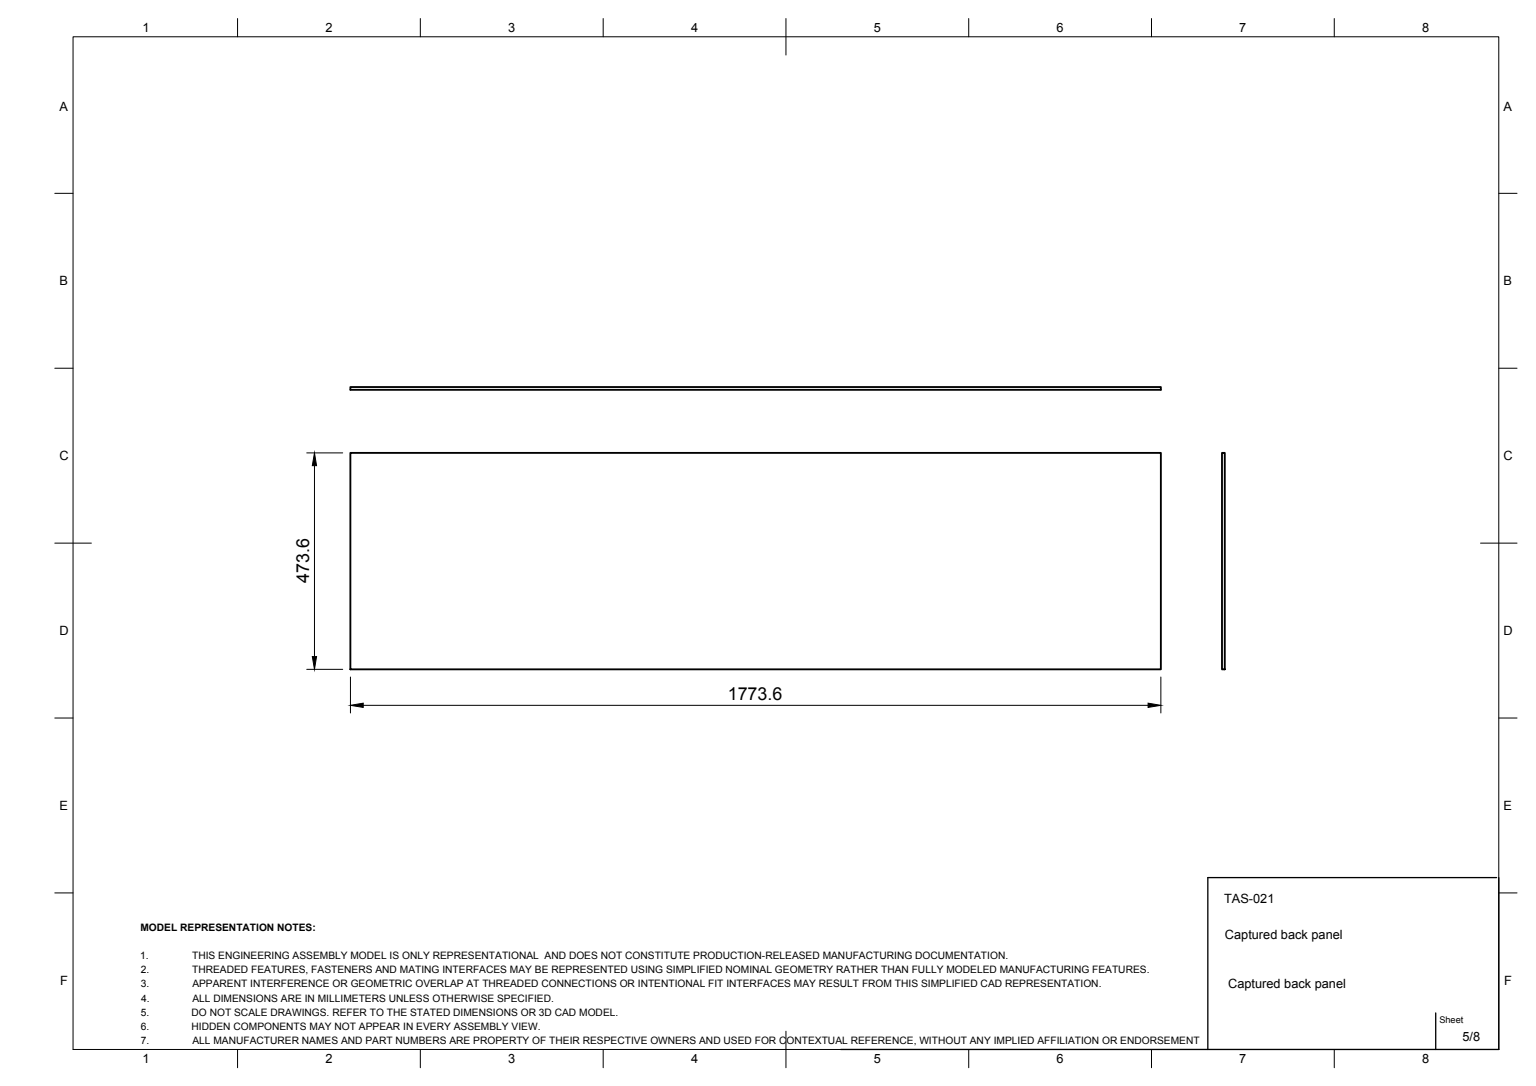
ISO-10303-21;
HEADER;
/* Generated by software containing ST-Developer
 * from STEP Tools, Inc. (www.steptools.com) 
 */

FILE_DESCRIPTION(
/* description */ (''),
/* implementation_level */ '2;1');

FILE_NAME(
/* name */ 'Captured back panel.step',
/* time_stamp */ '2026-11-15T17:48:08-08:00',
/* author */ (''),
/* organization */ (''),
/* preprocessor_version */ 'ST-DEVELOPER v20.2',
/* originating_system */ 'Autodesk Translation Framework v15.17.0.0',
/* authorisation */ '');

FILE_SCHEMA (('AUTOMOTIVE_DESIGN { 1 0 10303 214 3 1 1 }'));
ENDSEC;

DATA;
#10=MECHANICAL_DESIGN_GEOMETRIC_PRESENTATION_REPRESENTATION('',(#141),#2097);
#129=SHAPE_REPRESENTATION_RELATIONSHIP('SRR','None',#2148,#135);
#135=ADVANCED_BREP_SHAPE_REPRESENTATION('',(#147),#2093);
#141=STYLED_ITEM('',(#2187),#147);
#147=MANIFOLD_SOLID_BREP('Body1',#1195);
#197=PLANE('',#1326);
#198=PLANE('',#1327);
#199=PLANE('',#1328);
#200=PLANE('',#1329);
#201=PLANE('',#1330);
#202=PLANE('',#1331);
#259=FACE_OUTER_BOUND('',#331,.T.);
#260=FACE_OUTER_BOUND('',#332,.T.);
#261=FACE_OUTER_BOUND('',#333,.T.);
#262=FACE_OUTER_BOUND('',#334,.T.);
#263=FACE_OUTER_BOUND('',#335,.T.);
#264=FACE_OUTER_BOUND('',#336,.T.);
#331=EDGE_LOOP('',(#1045,#1046,#1047,#1048));
#332=EDGE_LOOP('',(#1049,#1050,#1051,#1052));
#333=EDGE_LOOP('',(#1053,#1054,#1055,#1056));
#334=EDGE_LOOP('',(#1057,#1058,#1059,#1060));
#335=EDGE_LOOP('',(#1061,#1062,#1063,#1064));
#336=EDGE_LOOP('',(#1065,#1066,#1067,#1068));
#445=LINE('',#1971,#563);
#446=LINE('',#1973,#564);
#447=LINE('',#1975,#565);
#448=LINE('',#1976,#566);
#449=LINE('',#1979,#567);
#450=LINE('',#1981,#568);
#451=LINE('',#1982,#569);
#452=LINE('',#1985,#570);
#453=LINE('',#1987,#571);
#454=LINE('',#1988,#572);
#455=LINE('',#1990,#573);
#456=LINE('',#1991,#574);
#563=VECTOR('',#1600,1.);
#564=VECTOR('',#1601,1.);
#565=VECTOR('',#1602,1.);
#566=VECTOR('',#1603,1.);
#567=VECTOR('',#1606,1.);
#568=VECTOR('',#1607,1.);
#569=VECTOR('',#1608,1.);
#570=VECTOR('',#1611,1.);
#571=VECTOR('',#1612,1.);
#572=VECTOR('',#1613,1.);
#573=VECTOR('',#1616,1.);
#574=VECTOR('',#1617,1.);
#679=VERTEX_POINT('',#1969);
#680=VERTEX_POINT('',#1970);
#681=VERTEX_POINT('',#1972);
#682=VERTEX_POINT('',#1974);
#683=VERTEX_POINT('',#1978);
#684=VERTEX_POINT('',#1980);
#685=VERTEX_POINT('',#1984);
#686=VERTEX_POINT('',#1986);
#805=EDGE_CURVE('',#679,#680,#445,.T.);
#806=EDGE_CURVE('',#680,#681,#446,.T.);
#807=EDGE_CURVE('',#682,#681,#447,.T.);
#808=EDGE_CURVE('',#679,#682,#448,.T.);
#809=EDGE_CURVE('',#683,#679,#449,.T.);
#810=EDGE_CURVE('',#684,#682,#450,.T.);
#811=EDGE_CURVE('',#683,#684,#451,.T.);
#812=EDGE_CURVE('',#685,#683,#452,.T.);
#813=EDGE_CURVE('',#686,#684,#453,.T.);
#814=EDGE_CURVE('',#685,#686,#454,.T.);
#815=EDGE_CURVE('',#680,#685,#455,.T.);
#816=EDGE_CURVE('',#681,#686,#456,.T.);
#1045=ORIENTED_EDGE('',*,*,#805,.T.);
#1046=ORIENTED_EDGE('',*,*,#806,.T.);
#1047=ORIENTED_EDGE('',*,*,#807,.F.);
#1048=ORIENTED_EDGE('',*,*,#808,.F.);
#1049=ORIENTED_EDGE('',*,*,#809,.T.);
#1050=ORIENTED_EDGE('',*,*,#808,.T.);
#1051=ORIENTED_EDGE('',*,*,#810,.F.);
#1052=ORIENTED_EDGE('',*,*,#811,.F.);
#1053=ORIENTED_EDGE('',*,*,#812,.T.);
#1054=ORIENTED_EDGE('',*,*,#811,.T.);
#1055=ORIENTED_EDGE('',*,*,#813,.F.);
#1056=ORIENTED_EDGE('',*,*,#814,.F.);
#1057=ORIENTED_EDGE('',*,*,#815,.T.);
#1058=ORIENTED_EDGE('',*,*,#814,.T.);
#1059=ORIENTED_EDGE('',*,*,#816,.F.);
#1060=ORIENTED_EDGE('',*,*,#806,.F.);
#1061=ORIENTED_EDGE('',*,*,#816,.T.);
#1062=ORIENTED_EDGE('',*,*,#813,.T.);
#1063=ORIENTED_EDGE('',*,*,#810,.T.);
#1064=ORIENTED_EDGE('',*,*,#807,.T.);
#1065=ORIENTED_EDGE('',*,*,#815,.F.);
#1066=ORIENTED_EDGE('',*,*,#805,.F.);
#1067=ORIENTED_EDGE('',*,*,#809,.F.);
#1068=ORIENTED_EDGE('',*,*,#812,.F.);
#1171=ADVANCED_FACE('',(#259),#197,.T.);
#1172=ADVANCED_FACE('',(#260),#198,.T.);
#1173=ADVANCED_FACE('',(#261),#199,.T.);
#1174=ADVANCED_FACE('',(#262),#200,.T.);
#1175=ADVANCED_FACE('',(#263),#201,.T.);
#1176=ADVANCED_FACE('',(#264),#202,.F.);
#1195=CLOSED_SHELL('',(#1171,#1172,#1173,#1174,#1175,#1176));
#1325=AXIS2_PLACEMENT_3D('',#1967,#1596,#1597);
#1326=AXIS2_PLACEMENT_3D('',#1968,#1598,#1599);
#1327=AXIS2_PLACEMENT_3D('',#1977,#1604,#1605);
#1328=AXIS2_PLACEMENT_3D('',#1983,#1609,#1610);
#1329=AXIS2_PLACEMENT_3D('',#1989,#1614,#1615);
#1330=AXIS2_PLACEMENT_3D('',#1992,#1618,#1619);
#1331=AXIS2_PLACEMENT_3D('',#1993,#1620,#1621);
#1596=DIRECTION('axis',(0.,0.,1.));
#1597=DIRECTION('refdir',(1.,0.,0.));
#1598=DIRECTION('center_axis',(0.,1.,0.));
#1599=DIRECTION('ref_axis',(-1.,0.,0.));
#1600=DIRECTION('',(-1.,0.,0.));
#1601=DIRECTION('',(0.,0.,1.));
#1602=DIRECTION('',(-1.,0.,0.));
#1603=DIRECTION('',(0.,0.,1.));
#1604=DIRECTION('center_axis',(1.,0.,0.));
#1605=DIRECTION('ref_axis',(0.,1.,0.));
#1606=DIRECTION('',(0.,1.,0.));
#1607=DIRECTION('',(0.,1.,0.));
#1608=DIRECTION('',(0.,0.,1.));
#1609=DIRECTION('center_axis',(0.,-1.,0.));
#1610=DIRECTION('ref_axis',(1.,0.,0.));
#1611=DIRECTION('',(1.,0.,0.));
#1612=DIRECTION('',(1.,0.,0.));
#1613=DIRECTION('',(0.,0.,1.));
#1614=DIRECTION('center_axis',(-1.,0.,0.));
#1615=DIRECTION('ref_axis',(0.,-1.,0.));
#1616=DIRECTION('',(0.,-1.,0.));
#1617=DIRECTION('',(0.,-1.,0.));
#1618=DIRECTION('center_axis',(0.,0.,1.));
#1619=DIRECTION('ref_axis',(1.,0.,0.));
#1620=DIRECTION('center_axis',(0.,0.,1.));
#1621=DIRECTION('ref_axis',(1.,0.,0.));
#1967=CARTESIAN_POINT('',(0.,0.,0.));
#1968=CARTESIAN_POINT('Origin',(47.36,0.6,0.));
#1969=CARTESIAN_POINT('',(47.36,0.6,0.));
#1970=CARTESIAN_POINT('',(0.,0.6,0.));
#1971=CARTESIAN_POINT('',(47.36,0.6,0.));
#1972=CARTESIAN_POINT('',(0.,0.6,177.36));
#1973=CARTESIAN_POINT('',(0.,0.6,0.));
#1974=CARTESIAN_POINT('',(47.36,0.6,177.36));
#1975=CARTESIAN_POINT('',(47.36,0.6,177.36));
#1976=CARTESIAN_POINT('',(47.36,0.6,0.));
#1977=CARTESIAN_POINT('Origin',(47.36,0.,0.));
#1978=CARTESIAN_POINT('',(47.36,0.,0.));
#1979=CARTESIAN_POINT('',(47.36,0.,0.));
#1980=CARTESIAN_POINT('',(47.36,0.,177.36));
#1981=CARTESIAN_POINT('',(47.36,0.,177.36));
#1982=CARTESIAN_POINT('',(47.36,0.,0.));
#1983=CARTESIAN_POINT('Origin',(0.,0.,0.));
#1984=CARTESIAN_POINT('',(0.,0.,0.));
#1985=CARTESIAN_POINT('',(0.,0.,0.));
#1986=CARTESIAN_POINT('',(0.,0.,177.36));
#1987=CARTESIAN_POINT('',(0.,0.,177.36));
#1988=CARTESIAN_POINT('',(0.,0.,0.));
#1989=CARTESIAN_POINT('Origin',(0.,0.6,0.));
#1990=CARTESIAN_POINT('',(0.,0.6,0.));
#1991=CARTESIAN_POINT('',(0.,0.6,177.36));
#1992=CARTESIAN_POINT('Origin',(23.68,0.3,177.36));
#1993=CARTESIAN_POINT('Origin',(23.68,0.3,0.));
#2085=UNCERTAINTY_MEASURE_WITH_UNIT(LENGTH_MEASURE(0.001),#2098,
'DISTANCE_ACCURACY_VALUE',
'Maximum model space distance between geometric entities at asserted c
onnectivities');
#2089=UNCERTAINTY_MEASURE_WITH_UNIT(LENGTH_MEASURE(0.001),#2098,
'DISTANCE_ACCURACY_VALUE',
'Maximum model space distance between geometric entities at asserted c
onnectivities');
#2093=(
GEOMETRIC_REPRESENTATION_CONTEXT(3)
GLOBAL_UNCERTAINTY_ASSIGNED_CONTEXT((#2085))
GLOBAL_UNIT_ASSIGNED_CONTEXT((#2098,#2100,#2101))
REPRESENTATION_CONTEXT('','3D')
);
#2097=(
GEOMETRIC_REPRESENTATION_CONTEXT(3)
GLOBAL_UNCERTAINTY_ASSIGNED_CONTEXT((#2089))
GLOBAL_UNIT_ASSIGNED_CONTEXT((#2098,#2100,#2101))
REPRESENTATION_CONTEXT('','3D')
);
#2098=(
LENGTH_UNIT()
NAMED_UNIT(*)
SI_UNIT(.CENTI.,.METRE.)
);
#2100=(
NAMED_UNIT(*)
PLANE_ANGLE_UNIT()
SI_UNIT($,.RADIAN.)
);
#2101=(
NAMED_UNIT(*)
SI_UNIT($,.STERADIAN.)
SOLID_ANGLE_UNIT()
);
#2105=SHAPE_DEFINITION_REPRESENTATION(#2112,#2148);
#2112=PRODUCT_DEFINITION_SHAPE('',$,#2156);
#2148=SHAPE_REPRESENTATION('',(#1325),#2093);
#2152=PRODUCT_DEFINITION_CONTEXT('part definition',#2175,'design');
#2156=PRODUCT_DEFINITION('Captured back panel','Captured back panel',#2163,
#2152);
#2163=PRODUCT_DEFINITION_FORMATION('',$,#2180);
#2175=APPLICATION_CONTEXT(
'Core Data for Automotive Mechanical Design Process');
#2176=PRODUCT_CONTEXT('part definition',#2175,'mechanical');
#2180=PRODUCT('Captured back panel','Captured back panel',$,(#2176));
#2187=PRESENTATION_STYLE_ASSIGNMENT((#2194));
#2194=SURFACE_STYLE_USAGE(.BOTH.,#2201);
#2201=SURFACE_SIDE_STYLE('',(#2208));
#2208=SURFACE_STYLE_FILL_AREA(#2215);
#2215=FILL_AREA_STYLE('Captured back panel finish',(#2222));
#2222=FILL_AREA_STYLE_COLOUR('Captured back panel finish',#2229);
#2229=COLOUR_RGB('Captured back panel finish',0.607843137254902,0.647058823529412,
0.701960784313725);
ENDSEC;
END-ISO-10303-21;
